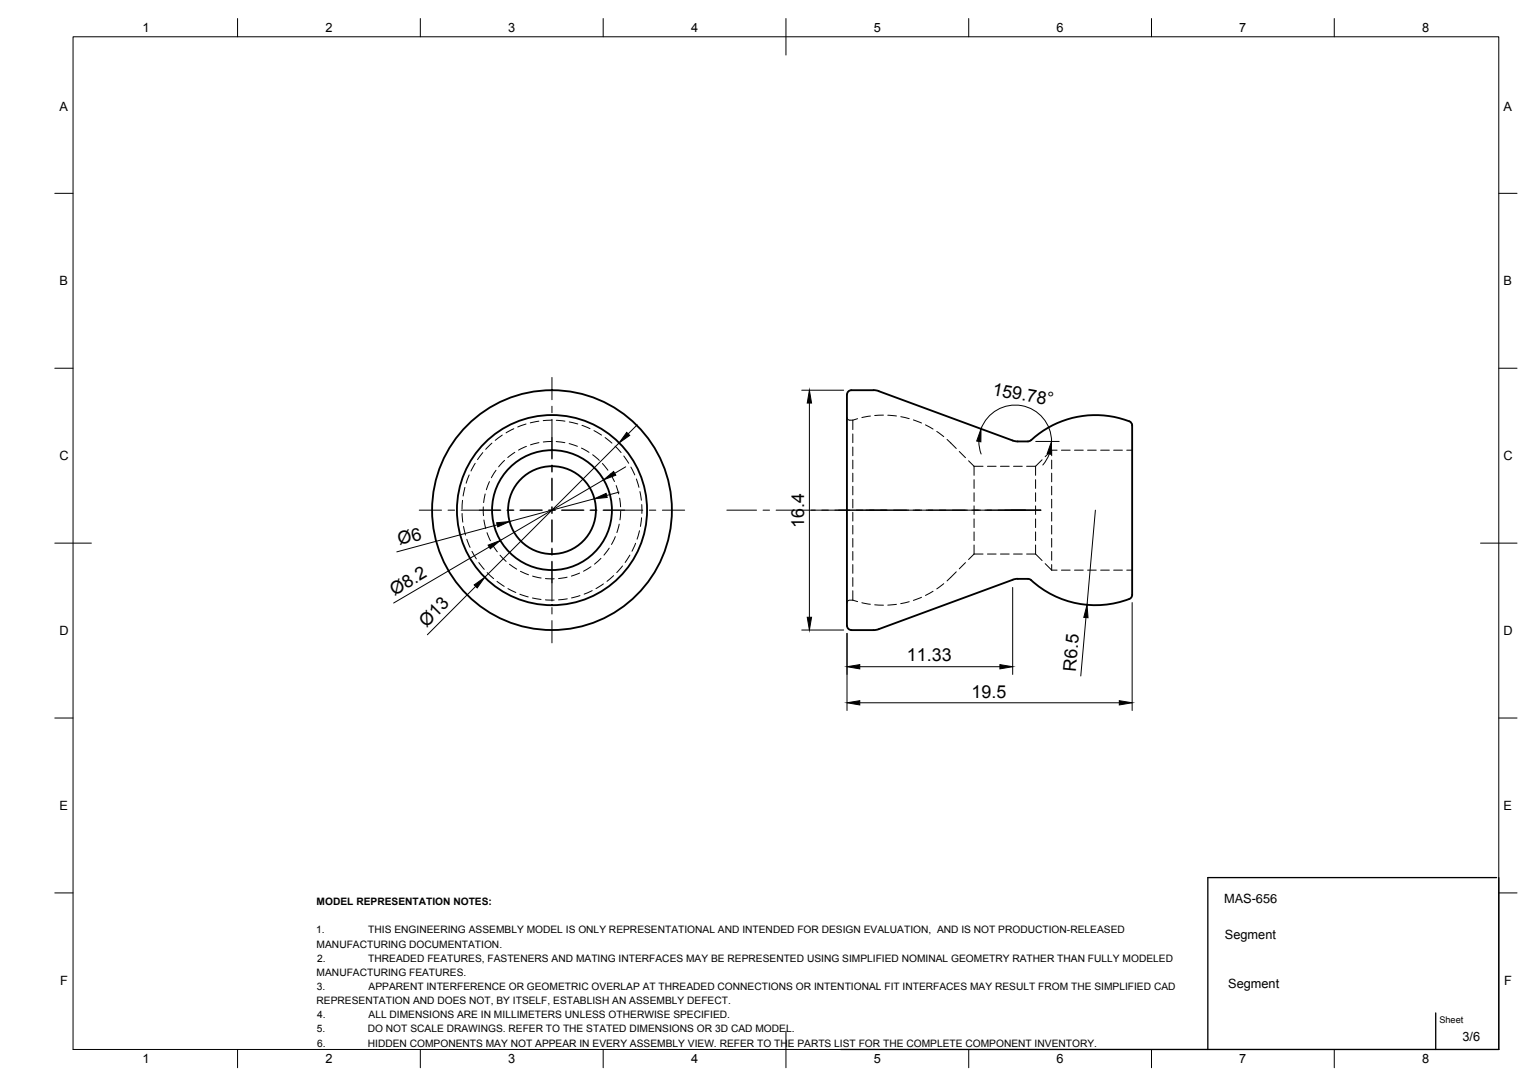
ISO-10303-21;
HEADER;
FILE_DESCRIPTION((''),'2;1');
FILE_NAME('Segment.step','2026-10-09T09:41:22-07:00',(''),(''),'','','');
FILE_SCHEMA (('AUTOMOTIVE_DESIGN { 1 0 10303 214 3 1 1 }'));
ENDSEC;
DATA;
#10=MECHANICAL_DESIGN_GEOMETRIC_PRESENTATION_REPRESENTATION('',(#78),#4304);
#68=SHAPE_REPRESENTATION_RELATIONSHIP('SRR','None',#4334,#72) ;
#72=ADVANCED_BREP_SHAPE_REPRESENTATION('',(#84),#4303) ;
#78=STYLED_ITEM('',(#4362),#84) ;
#84=MANIFOLD_SOLID_BREP('Body1',#2167) ;
#115=FACE_BOUND('',#770,.T.) ;
#116=FACE_BOUND('',#782,.T.) ;
#159=PLANE('',#2481) ;
#160=PLANE('',#2515) ;
#171=TOROIDAL_SURFACE('',#2483,5.7927412146,0.3) ;
#172=TOROIDAL_SURFACE('',#2491,5.,0.3) ;
#173=TOROIDAL_SURFACE('',#2498,5.7,1.) ;
#174=TOROIDAL_SURFACE('',#2502,7.9,0.3) ;
#175=TOROIDAL_SURFACE('',#2511,7.2,1.) ;
#176=TOROIDAL_SURFACE('',#2517,6.35142259969,0.2) ;
#218=CYLINDRICAL_SURFACE('',#2469,4.1) ;
#219=CYLINDRICAL_SURFACE('',#2474,3.) ;
#220=CYLINDRICAL_SURFACE('',#2495,4.7) ;
#221=CYLINDRICAL_SURFACE('',#2509,8.2) ;
#222=CYLINDRICAL_SURFACE('',#2513,6.15142259969) ;
#334=LINE('',#4204,#453) ;
#335=LINE('',#4209,#454) ;
#336=LINE('',#4213,#455) ;
#337=LINE('',#4216,#456) ;
#338=LINE('',#4245,#457) ;
#339=LINE('',#4266,#458) ;
#340=LINE('',#4270,#459) ;
#341=LINE('',#4276,#460) ;
#453=VECTOR('',#3157,4.1) ;
#454=VECTOR('',#3164,3.) ;
#455=VECTOR('',#3169,3.) ;
#456=VECTOR('',#3172,3.) ;
#457=VECTOR('',#3211,4.7) ;
#458=VECTOR('',#3238,4.7) ;
#459=VECTOR('',#3243,8.2) ;
#460=VECTOR('',#3252,6.15142259969) ;
#477=CONICAL_SURFACE('',#2472,3.,0.785398163397) ;
#478=CONICAL_SURFACE('',#2476,3.,0.785398163397) ;
#479=CONICAL_SURFACE('',#2507,4.7,0.352990387827) ;
#598=FACE_OUTER_BOUND('',#764,.T.) ;
#599=FACE_OUTER_BOUND('',#765,.T.) ;
#600=FACE_OUTER_BOUND('',#766,.T.) ;
#601=FACE_OUTER_BOUND('',#767,.T.) ;
#602=FACE_OUTER_BOUND('',#768,.T.) ;
#603=FACE_OUTER_BOUND('',#769,.T.) ;
#604=FACE_OUTER_BOUND('',#771,.T.) ;
#605=FACE_OUTER_BOUND('',#772,.T.) ;
#606=FACE_OUTER_BOUND('',#773,.T.) ;
#607=FACE_OUTER_BOUND('',#774,.T.) ;
#608=FACE_OUTER_BOUND('',#775,.T.) ;
#609=FACE_OUTER_BOUND('',#776,.T.) ;
#610=FACE_OUTER_BOUND('',#777,.T.) ;
#611=FACE_OUTER_BOUND('',#778,.T.) ;
#612=FACE_OUTER_BOUND('',#779,.T.) ;
#613=FACE_OUTER_BOUND('',#780,.T.) ;
#614=FACE_OUTER_BOUND('',#781,.T.) ;
#615=FACE_OUTER_BOUND('',#783,.T.) ;
#764=EDGE_LOOP('',(#1939,#1940,#1941,#1942)) ;
#765=EDGE_LOOP('',(#1943,#1944,#1945,#1946)) ;
#766=EDGE_LOOP('',(#1947,#1948,#1949,#1950)) ;
#767=EDGE_LOOP('',(#1951,#1952,#1953,#1954)) ;
#768=EDGE_LOOP('',(#1955,#1956,#1957,#1958)) ;
#769=EDGE_LOOP('',(#1959)) ;
#770=EDGE_LOOP('',(#1960)) ;
#771=EDGE_LOOP('',(#1961,#1962,#1963,#1964,#1965)) ;
#772=EDGE_LOOP('',(#1966,#1967,#1968,#1969,#1970,#1971)) ;
#773=EDGE_LOOP('',(#1972,#1973,#1974,#1975,#1976,#1977)) ;
#774=EDGE_LOOP('',(#1978,#1979,#1980,#1981,#1982,#1983)) ;
#775=EDGE_LOOP('',(#1984,#1985,#1986,#1987,#1988,#1989)) ;
#776=EDGE_LOOP('',(#1990,#1991,#1992,#1993,#1994)) ;
#777=EDGE_LOOP('',(#1995,#1996,#1997,#1998,#1999)) ;
#778=EDGE_LOOP('',(#2000,#2001,#2002,#2003,#2004)) ;
#779=EDGE_LOOP('',(#2005,#2006,#2007,#2008)) ;
#780=EDGE_LOOP('',(#2009,#2010,#2011,#2012)) ;
#781=EDGE_LOOP('',(#2013)) ;
#782=EDGE_LOOP('',(#2014)) ;
#783=EDGE_LOOP('',(#2015,#2016,#2017,#2018)) ;
#921=CIRCLE('',#2470,4.1) ;
#922=CIRCLE('',#2471,4.1) ;
#923=CIRCLE('',#2473,3.) ;
#924=CIRCLE('',#2475,3.) ;
#925=CIRCLE('',#2477,4.59619407771) ;
#926=CIRCLE('',#2479,6.15142259969) ;
#927=CIRCLE('',#2480,6.5) ;
#928=CIRCLE('',#2482,5.7927412146) ;
#929=CIRCLE('',#2484,0.3) ;
#930=CIRCLE('',#2485,6.07303514434) ;
#931=CIRCLE('',#2486,6.07303514434) ;
#932=CIRCLE('',#2488,6.5) ;
#933=CIRCLE('',#2489,4.77941176471) ;
#934=CIRCLE('',#2490,4.77941176471) ;
#935=CIRCLE('',#2492,0.3) ;
#936=CIRCLE('',#2493,4.7) ;
#937=CIRCLE('',#2494,4.7) ;
#938=CIRCLE('',#2496,4.7) ;
#939=CIRCLE('',#2497,4.7) ;
#940=CIRCLE('',#2499,1.) ;
#941=CIRCLE('',#2500,4.76165688318) ;
#942=CIRCLE('',#2501,4.76165688318) ;
#943=CIRCLE('',#2503,8.2) ;
#944=CIRCLE('',#2504,8.2) ;
#945=CIRCLE('',#2505,0.3) ;
#946=CIRCLE('',#2506,7.9) ;
#947=CIRCLE('',#2508,8.13834311682) ;
#948=CIRCLE('',#2510,8.2) ;
#949=CIRCLE('',#2512,1.) ;
#950=CIRCLE('',#2514,6.15142259969) ;
#951=CIRCLE('',#2516,6.35142259969) ;
#952=CIRCLE('',#2518,0.2) ;
#1113=VERTEX_POINT('',#4201) ;
#1114=VERTEX_POINT('',#4203) ;
#1115=VERTEX_POINT('',#4207) ;
#1116=VERTEX_POINT('',#4211) ;
#1117=VERTEX_POINT('',#4215) ;
#1118=VERTEX_POINT('',#4219) ;
#1119=VERTEX_POINT('',#4223) ;
#1120=VERTEX_POINT('',#4226) ;
#1121=VERTEX_POINT('',#4228) ;
#1122=VERTEX_POINT('',#4232) ;
#1123=VERTEX_POINT('',#4234) ;
#1124=VERTEX_POINT('',#4238) ;
#1125=VERTEX_POINT('',#4240) ;
#1126=VERTEX_POINT('',#4244) ;
#1127=VERTEX_POINT('',#4246) ;
#1128=VERTEX_POINT('',#4250) ;
#1129=VERTEX_POINT('',#4252) ;
#1130=VERTEX_POINT('',#4256) ;
#1131=VERTEX_POINT('',#4257) ;
#1132=VERTEX_POINT('',#4260) ;
#1133=VERTEX_POINT('',#4264) ;
#1134=VERTEX_POINT('',#4268) ;
#1135=VERTEX_POINT('',#4274) ;
#1136=VERTEX_POINT('',#4278) ;
#1391=EDGE_CURVE('',#1113,#1113,#921,.T.) ;
#1392=EDGE_CURVE('',#1113,#1114,#334,.T.) ;
#1393=EDGE_CURVE('',#1114,#1114,#922,.T.) ;
#1394=EDGE_CURVE('',#1115,#1115,#923,.T.) ;
#1395=EDGE_CURVE('',#1115,#1113,#335,.T.) ;
#1396=EDGE_CURVE('',#1116,#1116,#924,.T.) ;
#1397=EDGE_CURVE('',#1116,#1115,#336,.T.) ;
#1398=EDGE_CURVE('',#1116,#1117,#337,.T.) ;
#1399=EDGE_CURVE('',#1117,#1117,#925,.F.) ;
#1400=EDGE_CURVE('',#1118,#1118,#926,.T.) ;
#1401=EDGE_CURVE('',#1118,#1117,#927,.T.) ;
#1402=EDGE_CURVE('',#1119,#1119,#928,.T.) ;
#1403=EDGE_CURVE('',#1119,#1120,#929,.T.) ;
#1404=EDGE_CURVE('',#1120,#1121,#930,.T.) ;
#1405=EDGE_CURVE('',#1121,#1120,#931,.T.) ;
#1406=EDGE_CURVE('',#1121,#1122,#932,.T.) ;
#1407=EDGE_CURVE('',#1123,#1122,#933,.F.) ;
#1408=EDGE_CURVE('',#1122,#1123,#934,.F.) ;
#1409=EDGE_CURVE('',#1123,#1124,#935,.T.) ;
#1410=EDGE_CURVE('',#1125,#1124,#936,.F.) ;
#1411=EDGE_CURVE('',#1124,#1125,#937,.F.) ;
#1412=EDGE_CURVE('',#1125,#1126,#338,.T.) ;
#1413=EDGE_CURVE('',#1127,#1126,#938,.F.) ;
#1414=EDGE_CURVE('',#1126,#1127,#939,.F.) ;
#1415=EDGE_CURVE('',#1127,#1128,#940,.T.) ;
#1416=EDGE_CURVE('',#1129,#1128,#941,.F.) ;
#1417=EDGE_CURVE('',#1128,#1129,#942,.F.) ;
#1418=EDGE_CURVE('',#1130,#1131,#943,.T.) ;
#1419=EDGE_CURVE('',#1131,#1130,#944,.T.) ;
#1420=EDGE_CURVE('',#1131,#1132,#945,.T.) ;
#1421=EDGE_CURVE('',#1132,#1132,#946,.T.) ;
#1422=EDGE_CURVE('',#1133,#1133,#947,.F.) ;
#1423=EDGE_CURVE('',#1133,#1129,#339,.T.) ;
#1424=EDGE_CURVE('',#1134,#1134,#948,.T.) ;
#1425=EDGE_CURVE('',#1134,#1130,#340,.T.) ;
#1426=EDGE_CURVE('',#1134,#1133,#949,.T.) ;
#1427=EDGE_CURVE('',#1135,#1135,#950,.T.) ;
#1428=EDGE_CURVE('',#1135,#1118,#341,.T.) ;
#1429=EDGE_CURVE('',#1136,#1136,#951,.T.) ;
#1430=EDGE_CURVE('',#1136,#1135,#952,.T.) ;
#1939=ORIENTED_EDGE('',*,*,#1391,.F.) ;
#1940=ORIENTED_EDGE('',*,*,#1392,.T.) ;
#1941=ORIENTED_EDGE('',*,*,#1393,.T.) ;
#1942=ORIENTED_EDGE('',*,*,#1392,.F.) ;
#1943=ORIENTED_EDGE('',*,*,#1394,.F.) ;
#1944=ORIENTED_EDGE('',*,*,#1395,.T.) ;
#1945=ORIENTED_EDGE('',*,*,#1391,.T.) ;
#1946=ORIENTED_EDGE('',*,*,#1395,.F.) ;
#1947=ORIENTED_EDGE('',*,*,#1396,.F.) ;
#1948=ORIENTED_EDGE('',*,*,#1397,.T.) ;
#1949=ORIENTED_EDGE('',*,*,#1394,.T.) ;
#1950=ORIENTED_EDGE('',*,*,#1397,.F.) ;
#1951=ORIENTED_EDGE('',*,*,#1396,.T.) ;
#1952=ORIENTED_EDGE('',*,*,#1398,.T.) ;
#1953=ORIENTED_EDGE('',*,*,#1399,.F.) ;
#1954=ORIENTED_EDGE('',*,*,#1398,.F.) ;
#1955=ORIENTED_EDGE('',*,*,#1400,.F.) ;
#1956=ORIENTED_EDGE('',*,*,#1401,.T.) ;
#1957=ORIENTED_EDGE('',*,*,#1399,.T.) ;
#1958=ORIENTED_EDGE('',*,*,#1401,.F.) ;
#1959=ORIENTED_EDGE('',*,*,#1402,.T.) ;
#1960=ORIENTED_EDGE('',*,*,#1393,.F.) ;
#1961=ORIENTED_EDGE('',*,*,#1402,.F.) ;
#1962=ORIENTED_EDGE('',*,*,#1403,.T.) ;
#1963=ORIENTED_EDGE('',*,*,#1404,.T.) ;
#1964=ORIENTED_EDGE('',*,*,#1405,.T.) ;
#1965=ORIENTED_EDGE('',*,*,#1403,.F.) ;
#1966=ORIENTED_EDGE('',*,*,#1405,.F.) ;
#1967=ORIENTED_EDGE('',*,*,#1406,.T.) ;
#1968=ORIENTED_EDGE('',*,*,#1407,.F.) ;
#1969=ORIENTED_EDGE('',*,*,#1408,.F.) ;
#1970=ORIENTED_EDGE('',*,*,#1406,.F.) ;
#1971=ORIENTED_EDGE('',*,*,#1404,.F.) ;
#1972=ORIENTED_EDGE('',*,*,#1407,.T.) ;
#1973=ORIENTED_EDGE('',*,*,#1408,.T.) ;
#1974=ORIENTED_EDGE('',*,*,#1409,.T.) ;
#1975=ORIENTED_EDGE('',*,*,#1410,.F.) ;
#1976=ORIENTED_EDGE('',*,*,#1411,.F.) ;
#1977=ORIENTED_EDGE('',*,*,#1409,.F.) ;
#1978=ORIENTED_EDGE('',*,*,#1410,.T.) ;
#1979=ORIENTED_EDGE('',*,*,#1411,.T.) ;
#1980=ORIENTED_EDGE('',*,*,#1412,.T.) ;
#1981=ORIENTED_EDGE('',*,*,#1413,.F.) ;
#1982=ORIENTED_EDGE('',*,*,#1414,.F.) ;
#1983=ORIENTED_EDGE('',*,*,#1412,.F.) ;
#1984=ORIENTED_EDGE('',*,*,#1413,.T.) ;
#1985=ORIENTED_EDGE('',*,*,#1414,.T.) ;
#1986=ORIENTED_EDGE('',*,*,#1415,.T.) ;
#1987=ORIENTED_EDGE('',*,*,#1416,.F.) ;
#1988=ORIENTED_EDGE('',*,*,#1417,.F.) ;
#1989=ORIENTED_EDGE('',*,*,#1415,.F.) ;
#1990=ORIENTED_EDGE('',*,*,#1418,.F.) ;
#1991=ORIENTED_EDGE('',*,*,#1419,.F.) ;
#1992=ORIENTED_EDGE('',*,*,#1420,.T.) ;
#1993=ORIENTED_EDGE('',*,*,#1421,.T.) ;
#1994=ORIENTED_EDGE('',*,*,#1420,.F.) ;
#1995=ORIENTED_EDGE('',*,*,#1422,.T.) ;
#1996=ORIENTED_EDGE('',*,*,#1423,.T.) ;
#1997=ORIENTED_EDGE('',*,*,#1416,.T.) ;
#1998=ORIENTED_EDGE('',*,*,#1417,.T.) ;
#1999=ORIENTED_EDGE('',*,*,#1423,.F.) ;
#2000=ORIENTED_EDGE('',*,*,#1424,.F.) ;
#2001=ORIENTED_EDGE('',*,*,#1425,.T.) ;
#2002=ORIENTED_EDGE('',*,*,#1418,.T.) ;
#2003=ORIENTED_EDGE('',*,*,#1419,.T.) ;
#2004=ORIENTED_EDGE('',*,*,#1425,.F.) ;
#2005=ORIENTED_EDGE('',*,*,#1424,.T.) ;
#2006=ORIENTED_EDGE('',*,*,#1426,.T.) ;
#2007=ORIENTED_EDGE('',*,*,#1422,.F.) ;
#2008=ORIENTED_EDGE('',*,*,#1426,.F.) ;
#2009=ORIENTED_EDGE('',*,*,#1427,.F.) ;
#2010=ORIENTED_EDGE('',*,*,#1428,.T.) ;
#2011=ORIENTED_EDGE('',*,*,#1400,.T.) ;
#2012=ORIENTED_EDGE('',*,*,#1428,.F.) ;
#2013=ORIENTED_EDGE('',*,*,#1421,.F.) ;
#2014=ORIENTED_EDGE('',*,*,#1429,.T.) ;
#2015=ORIENTED_EDGE('',*,*,#1429,.F.) ;
#2016=ORIENTED_EDGE('',*,*,#1430,.T.) ;
#2017=ORIENTED_EDGE('',*,*,#1427,.T.) ;
#2018=ORIENTED_EDGE('',*,*,#1430,.F.) ;
#2024=SPHERICAL_SURFACE('',#2478,6.5) ;
#2025=SPHERICAL_SURFACE('',#2487,6.5) ;
#2144=ADVANCED_FACE('',(#598),#218,.F.) ;
#2145=ADVANCED_FACE('',(#599),#477,.F.) ;
#2146=ADVANCED_FACE('',(#600),#219,.F.) ;
#2147=ADVANCED_FACE('',(#601),#478,.F.) ;
#2148=ADVANCED_FACE('',(#602),#2024,.F.) ;
#2149=ADVANCED_FACE('',(#603,#115),#159,.T.) ;
#2150=ADVANCED_FACE('',(#604),#171,.T.) ;
#2151=ADVANCED_FACE('',(#605),#2025,.T.) ;
#2152=ADVANCED_FACE('',(#606),#172,.F.) ;
#2153=ADVANCED_FACE('',(#607),#220,.T.) ;
#2154=ADVANCED_FACE('',(#608),#173,.F.) ;
#2155=ADVANCED_FACE('',(#609),#174,.T.) ;
#2156=ADVANCED_FACE('',(#610),#479,.T.) ;
#2157=ADVANCED_FACE('',(#611),#221,.T.) ;
#2158=ADVANCED_FACE('',(#612),#175,.T.) ;
#2159=ADVANCED_FACE('',(#613),#222,.F.) ;
#2160=ADVANCED_FACE('',(#614,#116),#160,.F.) ;
#2161=ADVANCED_FACE('',(#615),#176,.T.) ;
#2167=CLOSED_SHELL('',(#2144,#2145,#2146,#2147,#2148,#2149,#2150,#2151,
#2152,#2153,#2154,#2155,#2156,#2157,#2158,#2159,#2160,#2161)) ;
#2468=AXIS2_PLACEMENT_3D('',#4199,#3151,#3152) ;
#2469=AXIS2_PLACEMENT_3D('',#4200,#3153,#3154) ;
#2470=AXIS2_PLACEMENT_3D('',#4202,#3155,#3156) ;
#2471=AXIS2_PLACEMENT_3D('',#4205,#3158,#3159) ;
#2472=AXIS2_PLACEMENT_3D('',#4206,#3160,#3161) ;
#2473=AXIS2_PLACEMENT_3D('',#4208,#3162,#3163) ;
#2474=AXIS2_PLACEMENT_3D('',#4210,#3165,#3166) ;
#2475=AXIS2_PLACEMENT_3D('',#4212,#3167,#3168) ;
#2476=AXIS2_PLACEMENT_3D('',#4214,#3170,#3171) ;
#2477=AXIS2_PLACEMENT_3D('',#4217,#3173,#3174) ;
#2478=AXIS2_PLACEMENT_3D('',#4218,#3175,#3176) ;
#2479=AXIS2_PLACEMENT_3D('',#4220,#3177,#3178) ;
#2480=AXIS2_PLACEMENT_3D('',#4221,#3179,#3180) ;
#2481=AXIS2_PLACEMENT_3D('',#4222,#3181,#3182) ;
#2482=AXIS2_PLACEMENT_3D('',#4224,#3183,#3184) ;
#2483=AXIS2_PLACEMENT_3D('',#4225,#3185,#3186) ;
#2484=AXIS2_PLACEMENT_3D('',#4227,#3187,#3188) ;
#2485=AXIS2_PLACEMENT_3D('',#4229,#3189,#3190) ;
#2486=AXIS2_PLACEMENT_3D('',#4230,#3191,#3192) ;
#2487=AXIS2_PLACEMENT_3D('',#4231,#3193,#3194) ;
#2488=AXIS2_PLACEMENT_3D('',#4233,#3195,#3196) ;
#2489=AXIS2_PLACEMENT_3D('',#4235,#3197,#3198) ;
#2490=AXIS2_PLACEMENT_3D('',#4236,#3199,#3200) ;
#2491=AXIS2_PLACEMENT_3D('',#4237,#3201,#3202) ;
#2492=AXIS2_PLACEMENT_3D('',#4239,#3203,#3204) ;
#2493=AXIS2_PLACEMENT_3D('',#4241,#3205,#3206) ;
#2494=AXIS2_PLACEMENT_3D('',#4242,#3207,#3208) ;
#2495=AXIS2_PLACEMENT_3D('',#4243,#3209,#3210) ;
#2496=AXIS2_PLACEMENT_3D('',#4247,#3212,#3213) ;
#2497=AXIS2_PLACEMENT_3D('',#4248,#3214,#3215) ;
#2498=AXIS2_PLACEMENT_3D('',#4249,#3216,#3217) ;
#2499=AXIS2_PLACEMENT_3D('',#4251,#3218,#3219) ;
#2500=AXIS2_PLACEMENT_3D('',#4253,#3220,#3221) ;
#2501=AXIS2_PLACEMENT_3D('',#4254,#3222,#3223) ;
#2502=AXIS2_PLACEMENT_3D('',#4255,#3224,#3225) ;
#2503=AXIS2_PLACEMENT_3D('',#4258,#3226,#3227) ;
#2504=AXIS2_PLACEMENT_3D('',#4259,#3228,#3229) ;
#2505=AXIS2_PLACEMENT_3D('',#4261,#3230,#3231) ;
#2506=AXIS2_PLACEMENT_3D('',#4262,#3232,#3233) ;
#2507=AXIS2_PLACEMENT_3D('',#4263,#3234,#3235) ;
#2508=AXIS2_PLACEMENT_3D('',#4265,#3236,#3237) ;
#2509=AXIS2_PLACEMENT_3D('',#4267,#3239,#3240) ;
#2510=AXIS2_PLACEMENT_3D('',#4269,#3241,#3242) ;
#2511=AXIS2_PLACEMENT_3D('',#4271,#3244,#3245) ;
#2512=AXIS2_PLACEMENT_3D('',#4272,#3246,#3247) ;
#2513=AXIS2_PLACEMENT_3D('',#4273,#3248,#3249) ;
#2514=AXIS2_PLACEMENT_3D('',#4275,#3250,#3251) ;
#2515=AXIS2_PLACEMENT_3D('',#4277,#3253,#3254) ;
#2516=AXIS2_PLACEMENT_3D('',#4279,#3255,#3256) ;
#2517=AXIS2_PLACEMENT_3D('',#4280,#3257,#3258) ;
#2518=AXIS2_PLACEMENT_3D('',#4281,#3259,#3260) ;
#3151=DIRECTION('axis',(0.,0.,1.)) ;
#3152=DIRECTION('refdir',(1.,0.,0.)) ;
#3153=DIRECTION('center_axis',(0.,-1.,0.)) ;
#3154=DIRECTION('ref_axis',(-0.479425538604203,0.,0.877582561890373)) ;
#3155=DIRECTION('center_axis',(0.,-1.,0.)) ;
#3156=DIRECTION('ref_axis',(0.,0.,1.)) ;
#3157=DIRECTION('',(0.,-1.,0.)) ;
#3158=DIRECTION('center_axis',(0.,-1.,0.)) ;
#3159=DIRECTION('ref_axis',(0.,0.,1.)) ;
#3160=DIRECTION('center_axis',(0.,-1.,0.)) ;
#3161=DIRECTION('ref_axis',(-0.479425538604204,0.,0.877582561890372)) ;
#3162=DIRECTION('center_axis',(0.,-1.,0.)) ;
#3163=DIRECTION('ref_axis',(0.,0.,1.)) ;
#3164=DIRECTION('',(0.339005049420894,-0.707106781186865,-0.620544580563467)) ;
#3165=DIRECTION('center_axis',(0.,-1.,0.)) ;
#3166=DIRECTION('ref_axis',(-0.479425538604204,0.,0.877582561890372)) ;
#3167=DIRECTION('center_axis',(0.,-1.,0.)) ;
#3168=DIRECTION('ref_axis',(0.,0.,1.)) ;
#3169=DIRECTION('',(0.,-1.,0.)) ;
#3170=DIRECTION('center_axis',(0.,1.,0.)) ;
#3171=DIRECTION('ref_axis',(-0.479425538604204,0.,0.877582561890372)) ;
#3172=DIRECTION('',(0.339005049420894,0.707106781186865,-0.620544580563467)) ;
#3173=DIRECTION('center_axis',(0.,1.,0.)) ;
#3174=DIRECTION('ref_axis',(0.,0.,-1.)) ;
#3175=DIRECTION('center_axis',(-8.80690426921701E-17,-1.,1.61209301310987E-16)) ;
#3176=DIRECTION('ref_axis',(-0.479425538604204,1.22464679914735E-16,0.877582561890372)) ;
#3177=DIRECTION('center_axis',(0.,-1.,0.)) ;
#3178=DIRECTION('ref_axis',(0.,0.,1.)) ;
#3179=DIRECTION('center_axis',(-0.877582561890372,-1.42222518970134E-31,
-0.479425538604204)) ;
#3180=DIRECTION('ref_axis',(0.479425538604204,-1.22464679914735E-16,-0.877582561890372)) ;
#3181=DIRECTION('center_axis',(0.,-1.,0.)) ;
#3182=DIRECTION('ref_axis',(1.,0.,0.)) ;
#3183=DIRECTION('center_axis',(0.,-1.,0.)) ;
#3184=DIRECTION('ref_axis',(0.,0.,1.)) ;
#3185=DIRECTION('center_axis',(0.,-1.,0.)) ;
#3186=DIRECTION('ref_axis',(0.136069885869001,0.,-0.990699241021006)) ;
#3187=DIRECTION('center_axis',(-0.990699241021006,0.,-0.136069885869001)) ;
#3188=DIRECTION('ref_axis',(-0.136069885869001,0.,0.990699241021006)) ;
#3189=DIRECTION('center_axis',(0.,-1.,0.)) ;
#3190=DIRECTION('ref_axis',(0.,0.,1.)) ;
#3191=DIRECTION('center_axis',(0.,-1.,0.)) ;
#3192=DIRECTION('ref_axis',(0.,0.,1.)) ;
#3193=DIRECTION('center_axis',(-8.80690426921701E-17,-1.,1.61209301310987E-16)) ;
#3194=DIRECTION('ref_axis',(-0.479425538604204,0.,0.877582561890372)) ;
#3195=DIRECTION('center_axis',(0.877582561890372,1.42222518970134E-31,0.479425538604204)) ;
#3196=DIRECTION('ref_axis',(0.479425538604204,0.,-0.877582561890372)) ;
#3197=DIRECTION('center_axis',(0.,-1.,0.)) ;
#3198=DIRECTION('ref_axis',(0.,0.,1.)) ;
#3199=DIRECTION('center_axis',(0.,-1.,0.)) ;
#3200=DIRECTION('ref_axis',(0.,0.,1.)) ;
#3201=DIRECTION('center_axis',(0.,-1.,0.)) ;
#3202=DIRECTION('ref_axis',(-0.127966679280044,0.,-0.991778467700342)) ;
#3203=DIRECTION('center_axis',(0.991778467700342,0.,-0.127966679280044)) ;
#3204=DIRECTION('ref_axis',(0.127966679280044,0.,0.991778467700342)) ;
#3205=DIRECTION('center_axis',(0.,-1.,0.)) ;
#3206=DIRECTION('ref_axis',(0.,0.,1.)) ;
#3207=DIRECTION('center_axis',(0.,-1.,0.)) ;
#3208=DIRECTION('ref_axis',(0.,0.,1.)) ;
#3209=DIRECTION('center_axis',(0.,-1.,0.)) ;
#3210=DIRECTION('ref_axis',(-0.479425538604204,0.,0.877582561890372)) ;
#3211=DIRECTION('',(0.,1.,0.)) ;
#3212=DIRECTION('center_axis',(0.,-1.,0.)) ;
#3213=DIRECTION('ref_axis',(0.,0.,1.)) ;
#3214=DIRECTION('center_axis',(0.,-1.,0.)) ;
#3215=DIRECTION('ref_axis',(0.,0.,1.)) ;
#3216=DIRECTION('center_axis',(0.,-1.,0.)) ;
#3217=DIRECTION('ref_axis',(-0.127966679280044,0.,-0.991778467700342)) ;
#3218=DIRECTION('center_axis',(0.991778467700342,0.,-0.127966679280044)) ;
#3219=DIRECTION('ref_axis',(0.127966679280044,0.,0.991778467700342)) ;
#3220=DIRECTION('center_axis',(0.,-1.,0.)) ;
#3221=DIRECTION('ref_axis',(0.,0.,1.)) ;
#3222=DIRECTION('center_axis',(0.,-1.,0.)) ;
#3223=DIRECTION('ref_axis',(0.,0.,1.)) ;
#3224=DIRECTION('center_axis',(0.,-1.,0.)) ;
#3225=DIRECTION('ref_axis',(0.405193516143217,0.,-0.91423094154349)) ;
#3226=DIRECTION('center_axis',(0.,-1.,0.)) ;
#3227=DIRECTION('ref_axis',(0.,0.,1.)) ;
#3228=DIRECTION('center_axis',(0.,-1.,0.)) ;
#3229=DIRECTION('ref_axis',(0.,0.,1.)) ;
#3230=DIRECTION('center_axis',(-0.91423094154349,0.,-0.405193516143217)) ;
#3231=DIRECTION('ref_axis',(-0.405193516143217,0.,0.91423094154349)) ;
#3232=DIRECTION('center_axis',(0.,-1.,0.)) ;
#3233=DIRECTION('ref_axis',(0.,0.,1.)) ;
#3234=DIRECTION('center_axis',(0.,1.,0.)) ;
#3235=DIRECTION('ref_axis',(-0.479425538604204,0.,0.877582561890372)) ;
#3236=DIRECTION('center_axis',(0.,1.,0.)) ;
#3237=DIRECTION('ref_axis',(0.,0.,-1.)) ;
#3238=DIRECTION('',(-0.165739977854205,-0.938343116817079,0.303384994459016)) ;
#3239=DIRECTION('center_axis',(0.,-1.,0.)) ;
#3240=DIRECTION('ref_axis',(-0.479425538604203,0.,0.877582561890373)) ;
#3241=DIRECTION('center_axis',(0.,-1.,0.)) ;
#3242=DIRECTION('ref_axis',(0.,0.,1.)) ;
#3243=DIRECTION('',(0.,1.,0.)) ;
#3244=DIRECTION('center_axis',(0.,1.,0.)) ;
#3245=DIRECTION('ref_axis',(-0.479425538604204,0.,0.877582561890372)) ;
#3246=DIRECTION('center_axis',(-0.877582561890372,0.,-0.479425538604204)) ;
#3247=DIRECTION('ref_axis',(0.479425538604204,0.,-0.877582561890372)) ;
#3248=DIRECTION('center_axis',(0.,-1.,0.)) ;
#3249=DIRECTION('ref_axis',(-0.479425538604204,0.,0.877582561890372)) ;
#3250=DIRECTION('center_axis',(0.,-1.,0.)) ;
#3251=DIRECTION('ref_axis',(0.,0.,1.)) ;
#3252=DIRECTION('',(0.,-1.,0.)) ;
#3253=DIRECTION('center_axis',(0.,-1.,0.)) ;
#3254=DIRECTION('ref_axis',(1.,0.,0.)) ;
#3255=DIRECTION('center_axis',(0.,-1.,0.)) ;
#3256=DIRECTION('ref_axis',(0.,0.,1.)) ;
#3257=DIRECTION('center_axis',(0.,-1.,0.)) ;
#3258=DIRECTION('ref_axis',(-0.479425538604204,0.,0.877582561890372)) ;
#3259=DIRECTION('center_axis',(0.877582561890372,0.,0.479425538604204)) ;
#3260=DIRECTION('ref_axis',(0.479425538604204,0.,-0.877582561890372)) ;
#4199=CARTESIAN_POINT('',(0.,0.,0.)) ;
#4200=CARTESIAN_POINT('Origin',(0.,-7.25000000007,0.)) ;
#4201=CARTESIAN_POINT('',(1.96564470827723,-11.5,-3.59808850375053)) ;
#4202=CARTESIAN_POINT('Origin',(0.,-11.5,0.)) ;
#4203=CARTESIAN_POINT('',(1.96564470827723,-17.,-3.59808850375053)) ;
#4204=CARTESIAN_POINT('',(1.96564470827723,-7.25000000007,-3.59808850375053)) ;
#4205=CARTESIAN_POINT('Origin',(0.,-17.,0.)) ;
#4206=CARTESIAN_POINT('Origin',(0.,-10.4,0.)) ;
#4207=CARTESIAN_POINT('',(1.43827661581261,-10.4,-2.63274768567112)) ;
#4208=CARTESIAN_POINT('Origin',(0.,-10.4,0.)) ;
#4209=CARTESIAN_POINT('',(1.43827661581261,-10.4,-2.63274768567112)) ;
#4210=CARTESIAN_POINT('Origin',(0.,-7.25000000007,0.)) ;
#4211=CARTESIAN_POINT('',(1.43827661581261,-6.19238815543,-2.63274768567112)) ;
#4212=CARTESIAN_POINT('Origin',(0.,-6.19238815543,0.)) ;
#4213=CARTESIAN_POINT('',(1.43827661581261,-7.25000000007,-2.63274768567112)) ;
#4214=CARTESIAN_POINT('Origin',(0.,-6.19238815543,0.)) ;
#4215=CARTESIAN_POINT('',(2.20353282123762,-4.59619407771428,-4.03353977366586)) ;
#4216=CARTESIAN_POINT('',(1.43827661581261,-6.19238815543,-2.63274768567112)) ;
#4217=CARTESIAN_POINT('Origin',(0.,-4.59619407771,0.)) ;
#4218=CARTESIAN_POINT('Origin',(0.,0.,0.)) ;
#4219=CARTESIAN_POINT('',(2.94914909303845,2.1,-5.39838120430629)) ;
#4220=CARTESIAN_POINT('Origin',(0.,2.1,0.)) ;
#4221=CARTESIAN_POINT('Origin',(0.,0.,0.)) ;
#4222=CARTESIAN_POINT('Origin',(0.,-17.,4.1)) ;
#4223=CARTESIAN_POINT('',(-0.788217635939279,-17.,5.73886432473532)) ;
#4224=CARTESIAN_POINT('Origin',(-8.881784197E-16,-17.,-1.7763568394E-15)) ;
#4225=CARTESIAN_POINT('Origin',(8.881784197E-16,-16.7,2.22044604925E-16)) ;
#4226=CARTESIAN_POINT('',(-0.826357198968776,-16.8069360227,6.01655130819153)) ;
#4227=CARTESIAN_POINT('Origin',(-0.78821763593928,-16.7,5.73886432473532)) ;
#4228=CARTESIAN_POINT('',(2.91156814503746,-16.8069360227,-5.32958974042017)) ;
#4229=CARTESIAN_POINT('Origin',(8.881784197E-16,-16.8069360227,2.22044604925E-16)) ;
#4230=CARTESIAN_POINT('Origin',(8.881784197E-16,-16.8069360227,2.22044604925E-16)) ;
#4231=CARTESIAN_POINT('Origin',(0.,-14.4899888641,5.93873487707E-17)) ;
#4232=CARTESIAN_POINT('',(2.29137205950736,-10.0846258617,-4.19432842080319)) ;
#4233=CARTESIAN_POINT('Origin',(0.,-14.4899888641,5.93873487707E-17)) ;
#4234=CARTESIAN_POINT('',(0.611605452441915,-10.0846258617,4.74011767651307)) ;
#4235=CARTESIAN_POINT('Origin',(0.,-10.0846258617,5.93873487707E-17)) ;
#4236=CARTESIAN_POINT('Origin',(0.,-10.0846258617,5.93873487707E-17)) ;
#4237=CARTESIAN_POINT('Origin',(1.11022302463E-15,-9.88130141541,4.4408920985E-16)) ;
#4238=CARTESIAN_POINT('',(0.601443392616207,-9.88130141541,4.66135879819161)) ;
#4239=CARTESIAN_POINT('Origin',(0.639833396400221,-9.88130141541,4.95889233850171)) ;
#4240=CARTESIAN_POINT('',(2.25330003143976,-9.88130141541,-4.12463804088475)) ;
#4241=CARTESIAN_POINT('Origin',(1.11022302463E-15,-9.88130141541,4.4408920985E-16)) ;
#4242=CARTESIAN_POINT('Origin',(1.11022302463E-15,-9.88130141541,4.4408920985E-16)) ;
#4243=CARTESIAN_POINT('Origin',(0.,-7.25000000007,0.)) ;
#4244=CARTESIAN_POINT('',(2.25330003143976,-9.17835096162,-4.12463804088475)) ;
#4245=CARTESIAN_POINT('',(2.25330003143976,-7.25000000007,-4.12463804088475)) ;
#4246=CARTESIAN_POINT('',(0.601443392616206,-9.17835096162,4.66135879819161)) ;
#4247=CARTESIAN_POINT('Origin',(0.,-9.17835096162,0.)) ;
#4248=CARTESIAN_POINT('Origin',(0.,-9.17835096162,0.)) ;
#4249=CARTESIAN_POINT('Origin',(-4.4408920985E-16,-9.17835096162,0.)) ;
#4250=CARTESIAN_POINT('',(0.609333419211508,-8.83264560279,4.72250876731505)) ;
#4251=CARTESIAN_POINT('Origin',(0.72941007189625,-9.17835096162,5.65313726589195)) ;
#4252=CARTESIAN_POINT('',(2.2828599158681,-8.83264560279086,-4.17874704638608)) ;
#4253=CARTESIAN_POINT('Origin',(-4.4408920985E-16,-8.83264560279,0.)) ;
#4254=CARTESIAN_POINT('Origin',(-4.4408920985E-16,-8.83264560279,0.)) ;
#4255=CARTESIAN_POINT('Origin',(1.7763568394E-15,2.2,8.881784197E-16)) ;
#4256=CARTESIAN_POINT('',(3.93128941655447,2.2,-7.19617700750105)) ;
#4257=CARTESIAN_POINT('',(-3.32258683237438,2.2,7.49669372065662)) ;
#4258=CARTESIAN_POINT('Origin',(-4.4408920985E-15,2.2,-2.6645352591E-15)) ;
#4259=CARTESIAN_POINT('Origin',(-4.4408920985E-15,2.2,-2.6645352591E-15)) ;
#4260=CARTESIAN_POINT('',(-3.20102877753141,2.5,7.22242443819357)) ;
#4261=CARTESIAN_POINT('Origin',(-3.20102877753141,2.2,7.22242443819357)) ;
#4262=CARTESIAN_POINT('Origin',(1.7763568394E-15,2.5,8.881784197E-16)) ;
#4263=CARTESIAN_POINT('Origin',(0.,-9.,0.)) ;
#4264=CARTESIAN_POINT('',(3.90172953212637,0.332645602789664,-7.14206800200019)) ;
#4265=CARTESIAN_POINT('Origin',(0.,0.332645602789,0.)) ;
#4266=CARTESIAN_POINT('',(2.25330003143976,-9.,-4.12463804088475)) ;
#4267=CARTESIAN_POINT('Origin',(0.,-7.25000000007,0.)) ;
#4268=CARTESIAN_POINT('',(3.93128941655,0.678350961617,-7.1961770075)) ;
#4269=CARTESIAN_POINT('Origin',(0.,0.678350961617,0.)) ;
#4270=CARTESIAN_POINT('',(3.93128941655446,-7.25000000007,-7.19617700750106)) ;
#4271=CARTESIAN_POINT('Origin',(4.4408920985E-16,0.678350961617,8.881784197E-16)) ;
#4272=CARTESIAN_POINT('Origin',(3.45186387795027,0.678350961617,-6.31859444561068)) ;
#4273=CARTESIAN_POINT('Origin',(0.,-7.25000000007,0.)) ;
#4274=CARTESIAN_POINT('',(2.94914909304,2.3,-5.39838120431)) ;
#4275=CARTESIAN_POINT('Origin',(0.,2.3,0.)) ;
#4276=CARTESIAN_POINT('',(2.94914909303845,-7.25000000007,-5.39838120430628)) ;
#4277=CARTESIAN_POINT('Origin',(0.,2.5,8.2)) ;
#4278=CARTESIAN_POINT('',(3.04503425308,2.5,-5.57389768811)) ;
#4279=CARTESIAN_POINT('Origin',(3.21964677141E-15,2.5,-5.3290705182E-15)) ;
#4280=CARTESIAN_POINT('Origin',(1.7763568394E-15,2.3,1.11022302463E-15)) ;
#4281=CARTESIAN_POINT('Origin',(3.0450342007593,2.3,-5.57389771668436)) ;
#4297=UNCERTAINTY_MEASURE_WITH_UNIT(LENGTH_MEASURE(0.01),#4305,
'DISTANCE_ACCURACY_VALUE',
'Maximum model space distance between geometric entities at asserted c
onnectivities') ;
#4298=UNCERTAINTY_MEASURE_WITH_UNIT(LENGTH_MEASURE(0.01),#4305,
'DISTANCE_ACCURACY_VALUE',
'Maximum model space distance between geometric entities at asserted c
onnectivities') ;
#4303=(
GEOMETRIC_REPRESENTATION_CONTEXT(3)
GLOBAL_UNCERTAINTY_ASSIGNED_CONTEXT((#4297))
GLOBAL_UNIT_ASSIGNED_CONTEXT((#4305,#4307,#4308))
REPRESENTATION_CONTEXT('','3D')
) ;
#4304=(
GEOMETRIC_REPRESENTATION_CONTEXT(3)
GLOBAL_UNCERTAINTY_ASSIGNED_CONTEXT((#4298))
GLOBAL_UNIT_ASSIGNED_CONTEXT((#4305,#4307,#4308))
REPRESENTATION_CONTEXT('','3D')
) ;
#4305=(
LENGTH_UNIT()
NAMED_UNIT(*)
SI_UNIT(.MILLI.,.METRE.)
) ;
#4307=(
NAMED_UNIT(*)
PLANE_ANGLE_UNIT()
SI_UNIT($,.RADIAN.)
) ;
#4308=(
NAMED_UNIT(*)
SI_UNIT($,.STERADIAN.)
SOLID_ANGLE_UNIT()
) ;
#4313=SHAPE_DEFINITION_REPRESENTATION(#4318,#4334) ;
#4318=PRODUCT_DEFINITION_SHAPE('',$,#4340) ;
#4334=SHAPE_REPRESENTATION('',(#2468),#4303) ;
#4335=PRODUCT_DEFINITION_CONTEXT('part definition',#4352,'design') ;
#4340=PRODUCT_DEFINITION('Segment','Segment',#4345,#4335) ;
#4345=PRODUCT_DEFINITION_FORMATION('',$,#4358) ;
#4352=APPLICATION_CONTEXT(
'Core Data for Automotive Mechanical Design Process') ;
#4353=PRODUCT_CONTEXT('part definition',#4352,'mechanical') ;
#4358=PRODUCT('Segment','Segment',$,(#4353)) ;
#4362=PRESENTATION_STYLE_ASSIGNMENT((#4366)) ;
#4366=SURFACE_STYLE_USAGE(.BOTH.,#4370) ;
#4370=SURFACE_SIDE_STYLE('',(#4374)) ;
#4374=SURFACE_STYLE_FILL_AREA(#4378) ;
#4378=FILL_AREA_STYLE('Opaque(48,59,150)',(#4382)) ;
#4382=FILL_AREA_STYLE_COLOUR('Opaque(48,59,150)',#4386) ;
#4386=COLOUR_RGB('Opaque(48,59,150)', 0.08235294, 0.09019608, 0.10196078) ;
ENDSEC;
END-ISO-10303-21;
